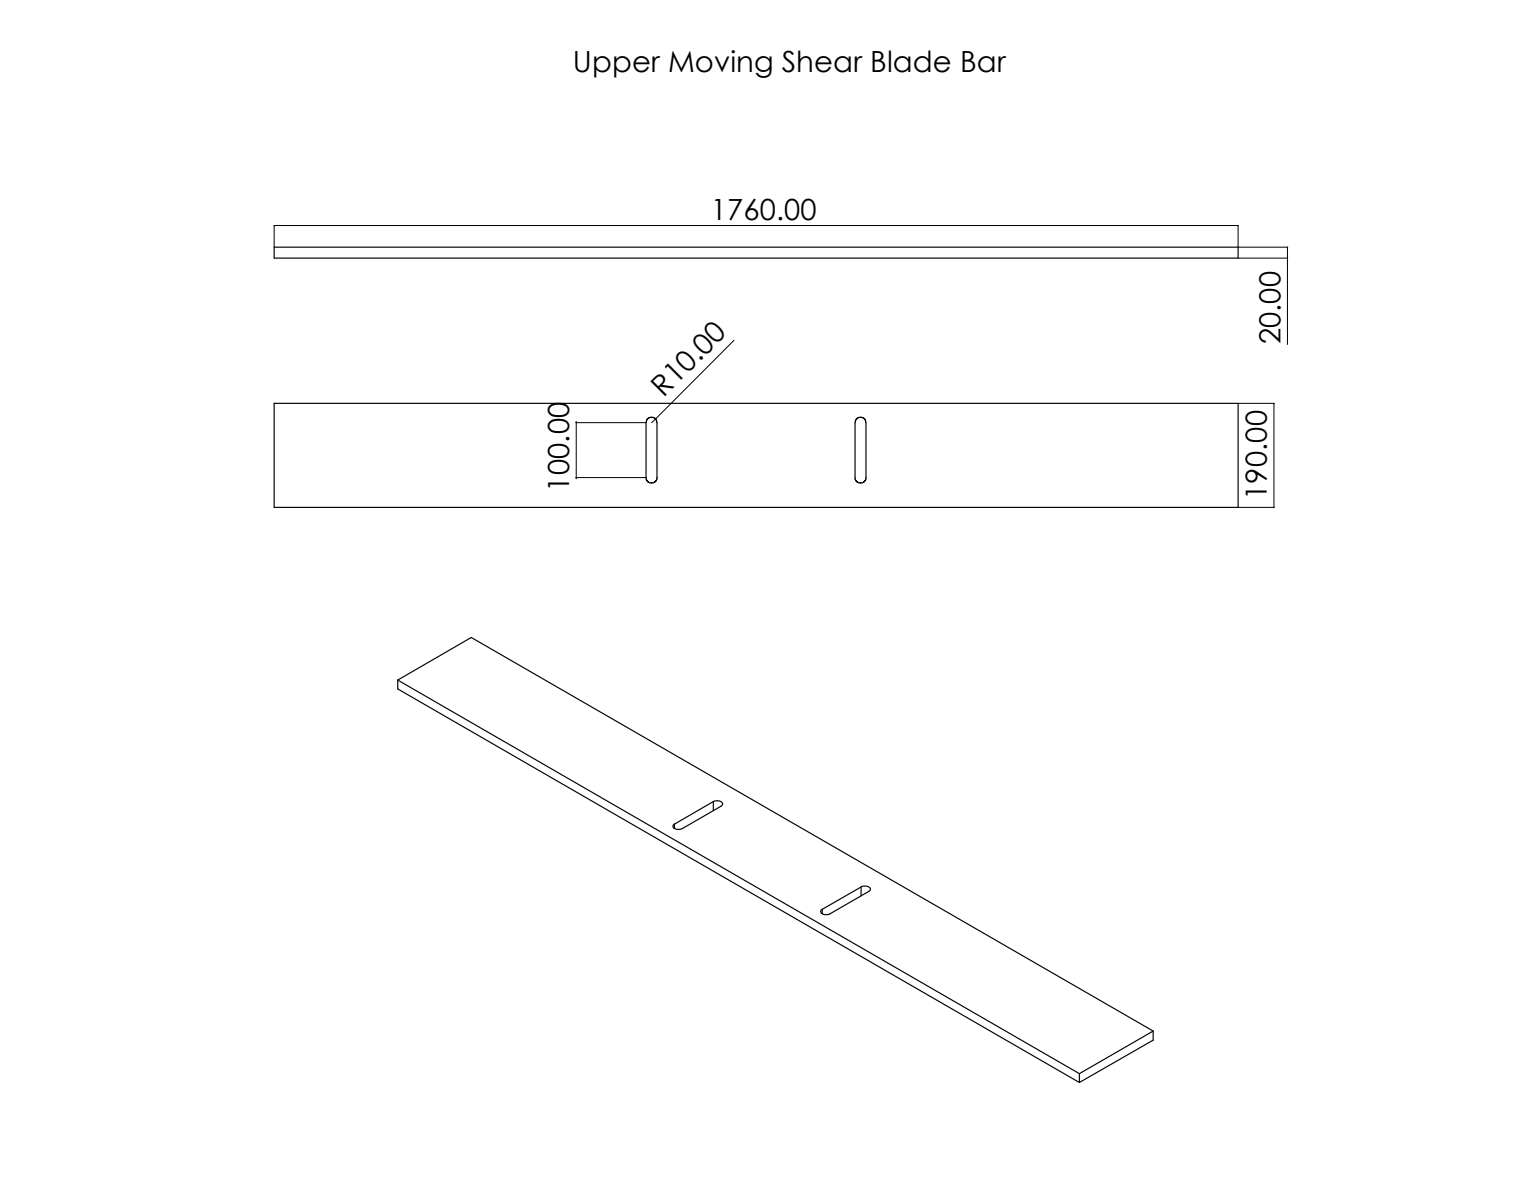
ISO-10303-21;
HEADER;
FILE_DESCRIPTION (('STEP AP214'),
    '1' );
FILE_NAME ('Upper Moving Shear Blade Bar.step',
    '2026-10-21T17:07:05',
    ( '' ),
    ( '' ),
    'SwSTEP 2.0',
    'SolidWorks 2025',
    '' );
FILE_SCHEMA (( 'AUTOMOTIVE_DESIGN' ));
ENDSEC;

DATA;
#27=ORIENTED_EDGE ( 'NONE', *, *, #22756, .F. ) ;
#29=LINE ( 'NONE', #5647, #43867 ) ;
#130=ORIENTED_EDGE ( 'NONE', *, *, #13131, .F. ) ;
#266=CARTESIAN_POINT ( 'NONE',  ( -180.7583438952258348, 394.6698570112193920, -224.9999999999999716 ) ) ;
#581=DIRECTION ( 'NONE',  ( 1.000000000000000000, -0.000000000000000000, 0.000000000000000000 ) ) ;
#901=DIRECTION ( 'NONE',  ( -1.000000000000000000, 1.892425610156518354E-16, 0.000000000000000000 ) ) ;
#935=DIRECTION ( 'NONE',  ( 1.000000000000000000, -8.326672684688676025E-16, 0.000000000000000000 ) ) ;
#1041=DIRECTION ( 'NONE',  ( -1.000000000000000000, 0.000000000000000000, 0.000000000000000000 ) ) ;
#1504=DIRECTION ( 'NONE',  ( 0.000000000000000000, 1.000000000000000000, 0.000000000000000000 ) ) ;
#1512=DIRECTION ( 'NONE',  ( 1.000000000000000000, 0.000000000000000000, -0.000000000000000000 ) ) ;
#1820=LINE ( 'NONE', #42339, #29283 ) ;
#1948=CARTESIAN_POINT ( 'NONE',  ( -190.7583438952259485, 394.6698570112193920, -274.9999999999999432 ) ) ;
#2119=LINE ( 'NONE', #11845, #11580 ) ;
#2127=FACE_OUTER_BOUND ( 'NONE', #44437, .T. ) ;
#2181=DIRECTION ( 'NONE',  ( 5.551115123125783688E-16, -1.000000000000000000, 0.000000000000000000 ) ) ;
#2576=EDGE_CURVE ( 'NONE', #42212, #45366, #43443, .T. ) ;
#2588=VECTOR ( 'NONE', #8913, 1000.000000000000000 ) ;
#2705=CARTESIAN_POINT ( 'NONE',  ( -180.7583438952258916, 294.6698570112193920, -224.9999999999999716 ) ) ;
#2814=ORIENTED_EDGE ( 'NONE', *, *, #20986, .T. ) ;
#2893=PLANE ( 'NONE',  #43166 ) ;
#2997=DIRECTION ( 'NONE',  ( 1.000000000000000000, 0.000000000000000000, 0.000000000000000000 ) ) ;
#3017=EDGE_CURVE ( 'NONE', #34587, #4508, #10696, .T. ) ;
#3213=ADVANCED_FACE ( 'NONE', ( #13857 ), #44817, .F. ) ;
#3240=VECTOR ( 'NONE', #38051, 1000.000000000000000 ) ;
#3278=DIRECTION ( 'NONE',  ( 8.326672684688676025E-16, -1.000000000000000000, 0.000000000000000000 ) ) ;
#3873=ORIENTED_EDGE ( 'NONE', *, *, #45007, .F. ) ;
#3881=PRODUCT_CONTEXT ( 'NONE', #32571, 'mechanical' ) ;
#3952=ADVANCED_BREP_SHAPE_REPRESENTATION ( '', ( #31868, #26858 ), #29006 ) ;
#4025=DIRECTION ( 'NONE',  ( -0.000000000000000000, -1.000000000000000000, -0.000000000000000000 ) ) ;
#4089=ADVANCED_FACE ( 'NONE', ( #39013 ), #14531, .F. ) ;
#4138=DIRECTION ( 'NONE',  ( -0.000000000000000000, -0.000000000000000000, 1.000000000000000000 ) ) ;
#4341=VERTEX_POINT ( 'NONE', #41669 ) ;
#4508=VERTEX_POINT ( 'NONE', #15438 ) ;
#4526=CARTESIAN_POINT ( 'NONE',  ( 200.7583438952258916, 294.6698570112193920, -274.9999999999999432 ) ) ;
#4681=DIRECTION ( 'NONE',  ( 1.000000000000000000, 0.000000000000000000, 0.000000000000000000 ) ) ;
#4964=EDGE_CURVE ( 'NONE', #45518, #8411, #15757, .T. ) ;
#5036=FACE_OUTER_BOUND ( 'NONE', #40726, .T. ) ;
#5163=ORIENTED_EDGE ( 'NONE', *, *, #18237, .F. ) ;
#5231=EDGE_LOOP ( 'NONE', ( #30202, #34802, #39527, #43738 ) ) ;
#5481=CIRCLE ( 'NONE', #32035, 10.00000000000006395 ) ;
#5489=VECTOR ( 'NONE', #4025, 1000.000000000000000 ) ;
#5504=EDGE_LOOP ( 'NONE', ( #24647, #14112, #14964, #44075 ) ) ;
#5520=DIRECTION ( 'NONE',  ( 1.000000000000000000, 0.000000000000000000, 0.000000000000000000 ) ) ;
#5588=STYLED_ITEM('',(#45779),#31868);
#5647=CARTESIAN_POINT ( 'NONE',  ( -200.7583438952257211, -1.114432678890474281E-13, -244.9999999999999716 ) ) ;
#5741=DIRECTION ( 'NONE',  ( 0.000000000000000000, -0.000000000000000000, 1.000000000000000000 ) ) ;
#5742=ORIENTED_EDGE ( 'NONE', *, *, #13885, .F. ) ;
#5789=EDGE_CURVE ( 'NONE', #17118, #17174, #27051, .T. ) ;
#5889=CARTESIAN_POINT ( 'NONE',  ( 200.7583438952259485, 394.6698570112193920, -274.9999999999999432 ) ) ;
#6035=ORIENTED_EDGE ( 'NONE', *, *, #39430, .F. ) ;
#6063=ORIENTED_EDGE ( 'NONE', *, *, #44462, .F. ) ;
#6075=DIRECTION ( 'NONE',  ( 1.000000000000000000, 0.000000000000000000, 0.000000000000000000 ) ) ;
#6252=AXIS2_PLACEMENT_3D ( 'NONE', #39369, #28745, #7499 ) ;
#6592=ORIENTED_EDGE ( 'NONE', *, *, #10942, .F. ) ;
#6658=EDGE_CURVE ( 'NONE', #34587, #37957, #36334, .T. ) ;
#6685=DIRECTION ( 'NONE',  ( 0.000000000000000000, -0.000000000000000000, 1.000000000000000000 ) ) ;
#6725=DIRECTION ( 'NONE',  ( -0.000000000000000000, -0.000000000000000000, 1.000000000000000000 ) ) ;
#6869=EDGE_LOOP ( 'NONE', ( #38404, #20507, #32932, #20169 ) ) ;
#6900=AXIS2_PLACEMENT_3D ( 'NONE', #21973, #935, #38668 ) ;
#7105=EDGE_LOOP ( 'NONE', ( #40674, #23927, #10024, #9838 ) ) ;
#7211=LINE ( 'NONE', #21284, #10700 ) ;
#7499=DIRECTION ( 'NONE',  ( 1.000000000000000000, 0.000000000000000000, 0.000000000000000000 ) ) ;
#7822=EDGE_CURVE ( 'NONE', #36156, #45518, #7211, .T. ) ;
#8396=CIRCLE ( 'NONE', #31234, 10.00000000000006395 ) ;
#8411=VERTEX_POINT ( 'NONE', #41123 ) ;
#8451=LINE ( 'NONE', #5889, #44550 ) ;
#8491=CARTESIAN_POINT ( 'NONE',  ( 200.7583438952259485, 394.6698570112193920, -244.9999999999999716 ) ) ;
#8510=CIRCLE ( 'NONE', #24705, 10.00000000000006395 ) ;
#8620=ORIENTED_EDGE ( 'NONE', *, *, #2576, .T. ) ;
#8685=CARTESIAN_POINT ( 'NONE',  ( 180.7583438952258348, 394.6698570112193920, -224.9999999999999716 ) ) ;
#8754=VERTEX_POINT ( 'NONE', #8491 ) ;
#8774=VERTEX_POINT ( 'NONE', #33871 ) ;
#8816=ORIENTED_EDGE ( 'NONE', *, *, #3017, .T. ) ;
#8860=ORIENTED_EDGE ( 'NONE', *, *, #2576, .F. ) ;
#8913=DIRECTION ( 'NONE',  ( 0.000000000000000000, 1.000000000000000000, 0.000000000000000000 ) ) ;
#9055=FACE_BOUND ( 'NONE', #27483, .T. ) ;
#9209=VERTEX_POINT ( 'NONE', #39869 ) ;
#9376=EDGE_CURVE ( 'NONE', #37957, #42212, #21806, .T. ) ;
#9394=AXIS2_PLACEMENT_3D ( 'NONE', #36836, #36620, #43534 ) ;
#9555=VERTEX_POINT ( 'NONE', #19060 ) ;
#9838=ORIENTED_EDGE ( 'NONE', *, *, #39646, .T. ) ;
#9993=( NAMED_UNIT ( * ) SI_UNIT ( $, .STERADIAN. ) SOLID_ANGLE_UNIT ( ) );
#10024=ORIENTED_EDGE ( 'NONE', *, *, #30379, .F. ) ;
#10532=CARTESIAN_POINT ( 'NONE',  ( -879.9999999999992042, 240.0000000000002274, -244.9999999999999716 ) ) ;
#10661=VECTOR ( 'NONE', #11122, 1000.000000000000000 ) ;
#10696=CIRCLE ( 'NONE', #18094, 10.00000000000000888 ) ;
#10700=VECTOR ( 'NONE', #35362, 1000.000000000000000 ) ;
#10730=FACE_OUTER_BOUND ( 'NONE', #45277, .T. ) ;
#10747=ORIENTED_EDGE ( 'NONE', *, *, #40559, .F. ) ;
#10942=EDGE_CURVE ( 'NONE', #32232, #4341, #17468, .T. ) ;
#11122=DIRECTION ( 'NONE',  ( 8.326672684688676025E-16, 1.000000000000000000, -0.000000000000000000 ) ) ;
#11149=( NAMED_UNIT ( * ) SI_UNIT ( $, .STERADIAN. ) SOLID_ANGLE_UNIT ( ) );
#11296=VECTOR ( 'NONE', #26217, 1000.000000000000000 ) ;
#11383=ORIENTED_EDGE ( 'NONE', *, *, #44462, .T. ) ;
#11412=DIRECTION ( 'NONE',  ( -0.000000000000000000, -0.000000000000000000, 1.000000000000000000 ) ) ;
#11440=ORIENTED_EDGE ( 'NONE', *, *, #38278, .F. ) ;
#11516=MECHANICAL_DESIGN_GEOMETRIC_PRESENTATION_REPRESENTATION('',(#5588),#17411);
#11580=VECTOR ( 'NONE', #16207, 1000.000000000000000 ) ;
#11627=DIRECTION ( 'NONE',  ( 1.000000000000000000, -5.551115123125783688E-16, 0.000000000000000000 ) ) ;
#11670=ADVANCED_FACE ( 'NONE', ( #19125 ), #33213, .F. ) ;
#11782=EDGE_LOOP ( 'NONE', ( #12503, #43387, #23339, #34195 ) ) ;
#11832=( LENGTH_UNIT ( ) NAMED_UNIT ( * ) SI_UNIT ( .MILLI., .METRE. ) );
#11845=CARTESIAN_POINT ( 'NONE',  ( -879.9999999999992042, 240.0000000000002274, -244.9999999999999716 ) ) ;
#11923=LINE ( 'NONE', #15614, #2588 ) ;
#12056=PRODUCT_DEFINITION_FORMATION_WITH_SPECIFIED_SOURCE ( 'ANY', '', #21473, .NOT_KNOWN. ) ;
#12153=VECTOR ( 'NONE', #14882, 1000.000000000000000 ) ;
#12380=FACE_BOUND ( 'NONE', #27839, .T. ) ;
#12503=ORIENTED_EDGE ( 'NONE', *, *, #17293, .T. ) ;
#12538=EDGE_CURVE ( 'NONE', #9209, #9555, #40081, .T. ) ;
#13131=EDGE_CURVE ( 'NONE', #4341, #27855, #26873, .T. ) ;
#13339=EDGE_CURVE ( 'NONE', #35556, #37602, #32944, .T. ) ;
#13644=ORIENTED_EDGE ( 'NONE', *, *, #39646, .F. ) ;
#13656=ORIENTED_EDGE ( 'NONE', *, *, #18237, .T. ) ;
#13662=ORIENTED_EDGE ( 'NONE', *, *, #19046, .T. ) ;
#13762=VECTOR ( 'NONE', #19614, 1000.000000000000000 ) ;
#13821=EDGE_LOOP ( 'NONE', ( #11383, #13644, #6035, #34359 ) ) ;
#13822=VECTOR ( 'NONE', #17631, 1000.000000000000000 ) ;
#13857=FACE_OUTER_BOUND ( 'NONE', #5231, .T. ) ;
#13885=EDGE_CURVE ( 'NONE', #4508, #35556, #1820, .T. ) ;
#13911=LINE ( 'NONE', #35366, #39751 ) ;
#14064=ORIENTED_EDGE ( 'NONE', *, *, #21274, .F. ) ;
#14112=ORIENTED_EDGE ( 'NONE', *, *, #42969, .T. ) ;
#14140=VECTOR ( 'NONE', #34457, 1000.000000000000000 ) ;
#14164=VERTEX_POINT ( 'NONE', #40195 ) ;
#14466=DIRECTION ( 'NONE',  ( 0.000000000000000000, 0.000000000000000000, 1.000000000000000000 ) ) ;
#14475=CARTESIAN_POINT ( 'NONE',  ( 879.9999999999992042, 239.9999999999998863, -244.9999999999999716 ) ) ;
#14531=PLANE ( 'NONE',  #44652 ) ;
#14871=ADVANCED_FACE ( 'NONE', ( #5036 ), #33215, .T. ) ;
#14877=LINE ( 'NONE', #25712, #23876 ) ;
#14882=DIRECTION ( 'NONE',  ( -0.000000000000000000, -0.000000000000000000, 1.000000000000000000 ) ) ;
#14964=ORIENTED_EDGE ( 'NONE', *, *, #24944, .F. ) ;
#15080=ORIENTED_EDGE ( 'NONE', *, *, #13885, .T. ) ;
#15325=CARTESIAN_POINT ( 'NONE',  ( 879.9999999999992042, 429.9999999999999432, -224.9999999999999716 ) ) ;
#15377=ORIENTED_EDGE ( 'NONE', *, *, #38278, .T. ) ;
#15398=FACE_BOUND ( 'NONE', #24156, .T. ) ;
#15438=CARTESIAN_POINT ( 'NONE',  ( -180.7583438952258916, 294.6698570112193920, -244.9999999999999716 ) ) ;
#15562=CARTESIAN_POINT ( 'NONE',  ( 180.7583438952258348, 394.6698570112193920, -274.9999999999999432 ) ) ;
#15614=CARTESIAN_POINT ( 'NONE',  ( -879.9999999999992042, 240.0000000000002274, -244.9999999999999716 ) ) ;
#15757=LINE ( 'NONE', #15325, #30675 ) ;
#15973=AXIS2_PLACEMENT_3D ( 'NONE', #26377, #16206, #4681 ) ;
#16073=EDGE_LOOP ( 'NONE', ( #44536, #19765, #44906, #31596 ) ) ;
#16206=DIRECTION ( 'NONE',  ( 0.000000000000000000, 0.000000000000000000, 1.000000000000000000 ) ) ;
#16207=DIRECTION ( 'NONE',  ( -0.000000000000000000, -0.000000000000000000, 1.000000000000000000 ) ) ;
#16215=CARTESIAN_POINT ( 'NONE',  ( 0.000000000000000000, 0.000000000000000000, -224.9999999999999716 ) ) ;
#16361=ORIENTED_EDGE ( 'NONE', *, *, #9376, .F. ) ;
#16538=ORIENTED_EDGE ( 'NONE', *, *, #17293, .F. ) ;
#16714=ORIENTED_EDGE ( 'NONE', *, *, #45007, .T. ) ;
#16743=AXIS2_PLACEMENT_3D ( 'NONE', #29730, #43808, #40385 ) ;
#16824=ORIENTED_EDGE ( 'NONE', *, *, #13339, .F. ) ;
#17054=ADVANCED_FACE ( 'NONE', ( #43935, #9055, #2127 ), #23121, .T. ) ;
#17118=VERTEX_POINT ( 'NONE', #43706 ) ;
#17125=FACE_OUTER_BOUND ( 'NONE', #41293, .T. ) ;
#17174=VERTEX_POINT ( 'NONE', #19016 ) ;
#17293=EDGE_CURVE ( 'NONE', #45518, #9555, #20361, .T. ) ;
#17411=( GEOMETRIC_REPRESENTATION_CONTEXT ( 3 ) GLOBAL_UNCERTAINTY_ASSIGNED_CONTEXT ( ( #32911 ) ) GLOBAL_UNIT_ASSIGNED_CONTEXT ( ( #37939, #45108, #9993 ) ) REPRESENTATION_CONTEXT ( 'NONE', 'WORKASPACE' ) );
#17417=PRODUCT_DEFINITION_SHAPE ( 'NONE', 'NONE',  #44518 ) ;
#17429=PLANE ( 'NONE',  #6900 ) ;
#17468=CIRCLE ( 'NONE', #15973, 10.00000000000000888 ) ;
#17487=LINE ( 'NONE', #28557, #45401 ) ;
#17631=DIRECTION ( 'NONE',  ( -0.000000000000000000, -0.000000000000000000, 1.000000000000000000 ) ) ;
#17673=CARTESIAN_POINT ( 'NONE',  ( 879.9999999999992042, 239.9999999999998863, -244.9999999999999716 ) ) ;
#17721=LINE ( 'NONE', #34343, #33434 ) ;
#17749=ORIENTED_EDGE ( 'NONE', *, *, #7822, .T. ) ;
#18085=( NAMED_UNIT ( * ) PLANE_ANGLE_UNIT ( ) SI_UNIT ( $, .RADIAN. ) );
#18094=AXIS2_PLACEMENT_3D ( 'NONE', #27933, #6685, #30948 ) ;
#18237=EDGE_CURVE ( 'NONE', #45366, #8774, #8510, .T. ) ;
#18305=CARTESIAN_POINT ( 'NONE',  ( -200.7583438952259485, 394.6698570112193920, -244.9999999999999716 ) ) ;
#18374=FACE_OUTER_BOUND ( 'NONE', #7105, .T. ) ;
#18435=VERTEX_POINT ( 'NONE', #10532 ) ;
#18482=EDGE_CURVE ( 'NONE', #8774, #37957, #17487, .T. ) ;
#18558=DIRECTION ( 'NONE',  ( -1.000000000000000000, 1.892425610156518354E-16, 0.000000000000000000 ) ) ;
#18766=EDGE_CURVE ( 'NONE', #17174, #4341, #29464, .T. ) ;
#18950=AXIS2_PLACEMENT_3D ( 'NONE', #20983, #35079, #43391 ) ;
#19016=CARTESIAN_POINT ( 'NONE',  ( 200.7583438952258916, 294.6698570112193920, -244.9999999999999716 ) ) ;
#19046=EDGE_CURVE ( 'NONE', #37602, #34587, #29, .T. ) ;
#19060=CARTESIAN_POINT ( 'NONE',  ( 879.9999999999992042, 239.9999999999998863, -224.9999999999999716 ) ) ;
#19064=CARTESIAN_POINT ( 'NONE',  ( -190.7583438952259485, 394.6698570112193920, -244.9999999999999716 ) ) ;
#19086=ADVANCED_FACE ( 'NONE', ( #17125 ), #27747, .F. ) ;
#19125=FACE_OUTER_BOUND ( 'NONE', #6869, .T. ) ;
#19223=DIRECTION ( 'NONE',  ( 0.000000000000000000, 0.000000000000000000, -1.000000000000000000 ) ) ;
#19374=ORIENTED_EDGE ( 'NONE', *, *, #18482, .F. ) ;
#19492=DIRECTION ( 'NONE',  ( 0.000000000000000000, -0.000000000000000000, 1.000000000000000000 ) ) ;
#19500=DIRECTION ( 'NONE',  ( 1.000000000000000000, 0.000000000000000000, 0.000000000000000000 ) ) ;
#19614=DIRECTION ( 'NONE',  ( -0.000000000000000000, -0.000000000000000000, 1.000000000000000000 ) ) ;
#19738=PLANE ( 'NONE',  #9394 ) ;
#19765=ORIENTED_EDGE ( 'NONE', *, *, #18482, .T. ) ;
#20169=ORIENTED_EDGE ( 'NONE', *, *, #3017, .F. ) ;
#20361=LINE ( 'NONE', #34683, #14140 ) ;
#20444=CARTESIAN_POINT ( 'NONE',  ( 879.9999999999992042, 239.9999999999998863, -244.9999999999999716 ) ) ;
#20507=ORIENTED_EDGE ( 'NONE', *, *, #9376, .T. ) ;
#20518=ADVANCED_FACE ( 'NONE', ( #15398, #12380, #43551 ), #26457, .F. ) ;
#20563=PRODUCT_DEFINITION_CONTEXT ( 'detailed design', #38789, 'design' ) ;
#20649=CARTESIAN_POINT ( 'NONE',  ( 879.9999999999992042, 429.9999999999999432, -224.9999999999999716 ) ) ;
#20659=DIRECTION ( 'NONE',  ( -1.000000000000000000, 1.892425610156518601E-16, 0.000000000000000000 ) ) ;
#20706=CARTESIAN_POINT ( 'NONE',  ( -879.9999999999992042, 430.0000000000002842, -224.9999999999999716 ) ) ;
#20878=CARTESIAN_POINT ( 'NONE',  ( 879.9999999999992042, 239.9999999999998863, -244.9999999999999716 ) ) ;
#20983=CARTESIAN_POINT ( 'NONE',  ( 190.7583438952258916, 294.6698570112193920, -244.9999999999999716 ) ) ;
#20986=EDGE_CURVE ( 'NONE', #8411, #9209, #45626, .T. ) ;
#21034=ADVANCED_FACE ( 'NONE', ( #32442 ), #25258, .F. ) ;
#21192=ORIENTED_EDGE ( 'NONE', *, *, #28021, .T. ) ;
#21250=ADVANCED_FACE ( 'NONE', ( #10730 ), #38930, .F. ) ;
#21274=EDGE_CURVE ( 'NONE', #37602, #8774, #31958, .T. ) ;
#21284=CARTESIAN_POINT ( 'NONE',  ( -879.9999999999992042, 430.0000000000002842, -224.9999999999999716 ) ) ;
#21301=LINE ( 'NONE', #29092, #35871 ) ;
#21331=DIRECTION ( 'NONE',  ( 8.326672684688676025E-16, 1.000000000000000000, 0.000000000000000000 ) ) ;
#21386=CARTESIAN_POINT ( 'NONE',  ( 180.7583438952258348, 394.6698570112193920, -244.9999999999999716 ) ) ;
#21396=DIRECTION ( 'NONE',  ( 5.551115123125783688E-16, -1.000000000000000000, 0.000000000000000000 ) ) ;
#21473=PRODUCT ( 'Upper Moving Shear Blade Bar', 'Upper Moving Shear Blade Bar', '', ( #3881 ) ) ;
#21555=DIRECTION ( 'NONE',  ( 0.000000000000000000, 0.000000000000000000, 1.000000000000000000 ) ) ;
#21806=CIRCLE ( 'NONE', #27706, 10.00000000000000888 ) ;
#21973=CARTESIAN_POINT ( 'NONE',  ( -180.7583438952258348, 394.6698570112193920, -274.9999999999999432 ) ) ;
#22096=ADVANCED_FACE ( 'NONE', ( #28051 ), #2893, .F. ) ;
#22217=EDGE_LOOP ( 'NONE', ( #43972, #8620, #28755, #5742 ) ) ;
#22261=PLANE ( 'NONE',  #32282 ) ;
#22756=EDGE_CURVE ( 'NONE', #23583, #14164, #37016, .T. ) ;
#23121=PLANE ( 'NONE',  #25898 ) ;
#23153=CARTESIAN_POINT ( 'NONE',  ( 0.000000000000000000, 0.000000000000000000, 0.000000000000000000 ) ) ;
#23221=AXIS2_PLACEMENT_3D ( 'NONE', #1948, #6725, #19500 ) ;
#23299=LINE ( 'NONE', #37620, #13762 ) ;
#23339=ORIENTED_EDGE ( 'NONE', *, *, #20986, .F. ) ;
#23583=VERTEX_POINT ( 'NONE', #21386 ) ;
#23876=VECTOR ( 'NONE', #21555, 1000.000000000000000 ) ;
#23927=ORIENTED_EDGE ( 'NONE', *, *, #28021, .F. ) ;
#23931=CARTESIAN_POINT ( 'NONE',  ( 879.9999999999992042, 239.9999999999998863, -224.9999999999999716 ) ) ;
#23948=VECTOR ( 'NONE', #11412, 1000.000000000000000 ) ;
#24137=ORIENTED_EDGE ( 'NONE', *, *, #39430, .T. ) ;
#24156=EDGE_LOOP ( 'NONE', ( #15377, #34878, #36680, #27894 ) ) ;
#24529=EDGE_LOOP ( 'NONE', ( #10747, #130, #6592, #27288 ) ) ;
#24566=DIRECTION ( 'NONE',  ( -1.000000000000000000, 0.000000000000000000, 0.000000000000000000 ) ) ;
#24647=ORIENTED_EDGE ( 'NONE', *, *, #22756, .T. ) ;
#24705=AXIS2_PLACEMENT_3D ( 'NONE', #30943, #28096, #35257 ) ;
#24785=PLANE ( 'NONE',  #27257 ) ;
#24834=ORIENTED_EDGE ( 'NONE', *, *, #13339, .T. ) ;
#24944=EDGE_CURVE ( 'NONE', #17118, #32232, #23299, .T. ) ;
#25258=PLANE ( 'NONE',  #35040 ) ;
#25472=CARTESIAN_POINT ( 'NONE',  ( 200.7583438952259485, 394.6698570112193920, -274.9999999999999432 ) ) ;
#25712=CARTESIAN_POINT ( 'NONE',  ( -879.9999999999992042, 430.0000000000002842, -244.9999999999999716 ) ) ;
#25898=AXIS2_PLACEMENT_3D ( 'NONE', #16215, #37226, #26600 ) ;
#25942=DIRECTION ( 'NONE',  ( -0.000000000000000000, -0.000000000000000000, 1.000000000000000000 ) ) ;
#26205=VECTOR ( 'NONE', #25942, 1000.000000000000000 ) ;
#26217=DIRECTION ( 'NONE',  ( 8.326672684688676025E-16, -1.000000000000000000, 0.000000000000000000 ) ) ;
#26377=CARTESIAN_POINT ( 'NONE',  ( 190.7583438952258916, 294.6698570112193920, -224.9999999999999716 ) ) ;
#26457=PLANE ( 'NONE',  #34231 ) ;
#26600=DIRECTION ( 'NONE',  ( 1.000000000000000000, 0.000000000000000000, -0.000000000000000000 ) ) ;
#26858=AXIS2_PLACEMENT_3D ( 'NONE', #23153, #34241, #6075 ) ;
#26873=LINE ( 'NONE', #33359, #27021 ) ;
#26975=ADVANCED_FACE ( 'NONE', ( #34042 ), #19738, .F. ) ;
#27021=VECTOR ( 'NONE', #33590, 1000.000000000000000 ) ;
#27051=CIRCLE ( 'NONE', #18950, 10.00000000000000888 ) ;
#27257=AXIS2_PLACEMENT_3D ( 'NONE', #25472, #11627, #35874 ) ;
#27288=ORIENTED_EDGE ( 'NONE', *, *, #42969, .F. ) ;
#27327=CARTESIAN_POINT ( 'NONE',  ( -200.7583438952258916, 294.6698570112193920, -244.9999999999999716 ) ) ;
#27474=LINE ( 'NONE', #34858, #36099 ) ;
#27483=EDGE_LOOP ( 'NONE', ( #5163, #8860, #16361, #19374 ) ) ;
#27706=AXIS2_PLACEMENT_3D ( 'NONE', #32694, #14466, #1041 ) ;
#27747=CYLINDRICAL_SURFACE ( 'NONE', #23221, 10.00000000000006395 ) ;
#27839=EDGE_LOOP ( 'NONE', ( #15080, #24834, #13662, #8816 ) ) ;
#27855=VERTEX_POINT ( 'NONE', #36329 ) ;
#27894=ORIENTED_EDGE ( 'NONE', *, *, #5789, .T. ) ;
#27933=CARTESIAN_POINT ( 'NONE',  ( -190.7583438952258916, 294.6698570112193920, -244.9999999999999716 ) ) ;
#28021=EDGE_CURVE ( 'NONE', #39568, #36156, #14877, .T. ) ;
#28051=FACE_OUTER_BOUND ( 'NONE', #13821, .T. ) ;
#28096=DIRECTION ( 'NONE',  ( 0.000000000000000000, 0.000000000000000000, 1.000000000000000000 ) ) ;
#28157=DIRECTION ( 'NONE',  ( -0.000000000000000000, -0.000000000000000000, 1.000000000000000000 ) ) ;
#28527=DIRECTION ( 'NONE',  ( 0.000000000000000000, 0.000000000000000000, -1.000000000000000000 ) ) ;
#28557=CARTESIAN_POINT ( 'NONE',  ( -200.7583438952259485, 394.6698570112193920, -224.9999999999999716 ) ) ;
#28677=EDGE_CURVE ( 'NONE', #8754, #23583, #5481, .T. ) ;
#28724=LINE ( 'NONE', #32421, #39617 ) ;
#28745=DIRECTION ( 'NONE',  ( -0.000000000000000000, -0.000000000000000000, 1.000000000000000000 ) ) ;
#28755=ORIENTED_EDGE ( 'NONE', *, *, #34585, .F. ) ;
#29006=( GEOMETRIC_REPRESENTATION_CONTEXT ( 3 ) GLOBAL_UNCERTAINTY_ASSIGNED_CONTEXT ( ( #34873 ) ) GLOBAL_UNIT_ASSIGNED_CONTEXT ( ( #11832, #18085, #11149 ) ) REPRESENTATION_CONTEXT ( 'NONE', 'WORKASPACE' ) );
#29092=CARTESIAN_POINT ( 'NONE',  ( 879.9999999999992042, 429.9999999999999432, -244.9999999999999716 ) ) ;
#29128=CLOSED_SHELL ( 'NONE', ( #21034, #22096, #33971, #20518, #17054, #14871, #19086, #43542, #11670, #4089, #21250, #39277, #3213, #26975 ) ) ;
#29272=ORIENTED_EDGE ( 'NONE', *, *, #13131, .T. ) ;
#29283=VECTOR ( 'NONE', #21331, 1000.000000000000000 ) ;
#29285=AXIS2_PLACEMENT_3D ( 'NONE', #35759, #4138, #32306 ) ;
#29464=LINE ( 'NONE', #4526, #33555 ) ;
#29691=CARTESIAN_POINT ( 'NONE',  ( 0.000000000000000000, 0.000000000000000000, -244.9999999999999716 ) ) ;
#29730=CARTESIAN_POINT ( 'NONE',  ( 8.137430123673030402E-14, 430.0000000000000568, 0.000000000000000000 ) ) ;
#29994=DIRECTION ( 'NONE',  ( 1.000000000000000000, 0.000000000000000000, 0.000000000000000000 ) ) ;
#30035=CARTESIAN_POINT ( 'NONE',  ( -200.7583438952258916, 294.6698570112193920, -224.9999999999999716 ) ) ;
#30202=ORIENTED_EDGE ( 'NONE', *, *, #24944, .T. ) ;
#30379=EDGE_CURVE ( 'NONE', #18435, #39568, #11923, .T. ) ;
#30675=VECTOR ( 'NONE', #19223, 1000.000000000000000 ) ;
#30718=AXIS2_PLACEMENT_3D ( 'NONE', #19064, #19492, #43982 ) ;
#30943=CARTESIAN_POINT ( 'NONE',  ( -190.7583438952259485, 394.6698570112193920, -224.9999999999999716 ) ) ;
#30948=DIRECTION ( 'NONE',  ( 1.000000000000000000, 0.000000000000000000, 0.000000000000000000 ) ) ;
#30969=CARTESIAN_POINT ( 'NONE',  ( -180.7583438952258348, 394.6698570112193920, -244.9999999999999716 ) ) ;
#31234=AXIS2_PLACEMENT_3D ( 'NONE', #35568, #32359, #5520 ) ;
#31596=ORIENTED_EDGE ( 'NONE', *, *, #19046, .F. ) ;
#31735=DIRECTION ( 'NONE',  ( 0.000000000000000000, 0.000000000000000000, 1.000000000000000000 ) ) ;
#31868=MANIFOLD_SOLID_BREP ( 'Cut-Extrude5[2]', #29128 ) ;
#31958=LINE ( 'NONE', #43050, #23948 ) ;
#32035=AXIS2_PLACEMENT_3D ( 'NONE', #33456, #5741, #29994 ) ;
#32167=SHAPE_REPRESENTATION_RELATIONSHIP ( 'NONE' , 'NONE' ,  #36841, #3952 ) ;
#32168=VECTOR ( 'NONE', #35697, 1000.000000000000000 ) ;
#32221=CARTESIAN_POINT ( 'NONE',  ( -879.9999999999992042, 240.0000000000002274, -244.9999999999999716 ) ) ;
#32232=VERTEX_POINT ( 'NONE', #43622 ) ;
#32282=AXIS2_PLACEMENT_3D ( 'NONE', #32221, #581, #28527 ) ;
#32302=DIRECTION ( 'NONE',  ( 5.551115123125783688E-16, -1.000000000000000000, 0.000000000000000000 ) ) ;
#32306=DIRECTION ( 'NONE',  ( 1.000000000000000000, 0.000000000000000000, 0.000000000000000000 ) ) ;
#32345=EDGE_CURVE ( 'NONE', #8411, #39568, #21301, .T. ) ;
#32359=DIRECTION ( 'NONE',  ( 0.000000000000000000, 0.000000000000000000, 1.000000000000000000 ) ) ;
#32421=CARTESIAN_POINT ( 'NONE',  ( 879.9999999999992042, 239.9999999999998863, -244.9999999999999716 ) ) ;
#32433=CARTESIAN_POINT ( 'NONE',  ( -200.7583438952258916, 294.6698570112193920, -274.9999999999999432 ) ) ;
#32442=FACE_OUTER_BOUND ( 'NONE', #11782, .T. ) ;
#32571=APPLICATION_CONTEXT ( 'automotive_design' ) ;
#32694=CARTESIAN_POINT ( 'NONE',  ( -190.7583438952258916, 294.6698570112193920, -224.9999999999999716 ) ) ;
#32911=UNCERTAINTY_MEASURE_WITH_UNIT (LENGTH_MEASURE( 1.000000000000000082E-05 ), #37939, 'distance_accuracy_value', 'NONE');
#32932=ORIENTED_EDGE ( 'NONE', *, *, #44199, .F. ) ;
#32944=CIRCLE ( 'NONE', #30718, 10.00000000000006395 ) ;
#33168=CARTESIAN_POINT ( 'NONE',  ( -879.9999999999992042, 240.0000000000002274, -224.9999999999999716 ) ) ;
#33213=CYLINDRICAL_SURFACE ( 'NONE', #29285, 10.00000000000000888 ) ;
#33215=PLANE ( 'NONE',  #16743 ) ;
#33359=CARTESIAN_POINT ( 'NONE',  ( 200.7583438952259485, 394.6698570112193920, -224.9999999999999716 ) ) ;
#33365=DIRECTION ( 'NONE',  ( -0.000000000000000000, -0.000000000000000000, 1.000000000000000000 ) ) ;
#33434=VECTOR ( 'NONE', #37814, 1000.000000000000000 ) ;
#33456=CARTESIAN_POINT ( 'NONE',  ( 190.7583438952259485, 394.6698570112193920, -244.9999999999999716 ) ) ;
#33555=VECTOR ( 'NONE', #33365, 1000.000000000000000 ) ;
#33590=DIRECTION ( 'NONE',  ( 5.551115123125783688E-16, 1.000000000000000000, -0.000000000000000000 ) ) ;
#33871=CARTESIAN_POINT ( 'NONE',  ( -200.7583438952259485, 394.6698570112193920, -224.9999999999999716 ) ) ;
#33912=ORIENTED_EDGE ( 'NONE', *, *, #32345, .T. ) ;
#33971=ADVANCED_FACE ( 'NONE', ( #18374 ), #22261, .F. ) ;
#34042=FACE_OUTER_BOUND ( 'NONE', #5504, .T. ) ;
#34195=ORIENTED_EDGE ( 'NONE', *, *, #4964, .F. ) ;
#34231=AXIS2_PLACEMENT_3D ( 'NONE', #29691, #40558, #1512 ) ;
#34241=DIRECTION ( 'NONE',  ( 0.000000000000000000, 0.000000000000000000, 1.000000000000000000 ) ) ;
#34343=CARTESIAN_POINT ( 'NONE',  ( -180.7583438952258916, 294.6698570112193920, -274.9999999999999432 ) ) ;
#34359=ORIENTED_EDGE ( 'NONE', *, *, #12538, .T. ) ;
#34457=DIRECTION ( 'NONE',  ( -0.000000000000000000, -1.000000000000000000, -0.000000000000000000 ) ) ;
#34487=LINE ( 'NONE', #38639, #13822 ) ;
#34585=EDGE_CURVE ( 'NONE', #35556, #45366, #34487, .T. ) ;
#34587=VERTEX_POINT ( 'NONE', #27327 ) ;
#34640=CARTESIAN_POINT ( 'NONE',  ( 190.7583438952258916, 294.6698570112193920, -274.9999999999999432 ) ) ;
#34683=CARTESIAN_POINT ( 'NONE',  ( 879.9999999999992042, 239.9999999999998863, -224.9999999999999716 ) ) ;
#34802=ORIENTED_EDGE ( 'NONE', *, *, #10942, .T. ) ;
#34858=CARTESIAN_POINT ( 'NONE',  ( 200.7583438952257211, -1.114432678890474281E-13, -244.9999999999999716 ) ) ;
#34873=UNCERTAINTY_MEASURE_WITH_UNIT (LENGTH_MEASURE( 1.000000000000000082E-05 ), #11832, 'distance_accuracy_value', 'NONE');
#34878=ORIENTED_EDGE ( 'NONE', *, *, #28677, .T. ) ;
#34954=VECTOR ( 'NONE', #1504, 1000.000000000000000 ) ;
#35040=AXIS2_PLACEMENT_3D ( 'NONE', #17673, #24566, #31735 ) ;
#35079=DIRECTION ( 'NONE',  ( 0.000000000000000000, -0.000000000000000000, 1.000000000000000000 ) ) ;
#35257=DIRECTION ( 'NONE',  ( -1.000000000000000000, 0.000000000000000000, 0.000000000000000000 ) ) ;
#35362=DIRECTION ( 'NONE',  ( 1.000000000000000000, -1.892425610156518354E-16, 0.000000000000000000 ) ) ;
#35366=CARTESIAN_POINT ( 'NONE',  ( 180.7583438952261474, 1.505115564641941601E-13, -244.9999999999999716 ) ) ;
#35556=VERTEX_POINT ( 'NONE', #30969 ) ;
#35568=CARTESIAN_POINT ( 'NONE',  ( 190.7583438952259485, 394.6698570112193920, -224.9999999999999716 ) ) ;
#35697=DIRECTION ( 'NONE',  ( -0.000000000000000000, -0.000000000000000000, 1.000000000000000000 ) ) ;
#35759=CARTESIAN_POINT ( 'NONE',  ( -190.7583438952258916, 294.6698570112193920, -274.9999999999999432 ) ) ;
#35871=VECTOR ( 'NONE', #901, 1000.000000000000000 ) ;
#35874=DIRECTION ( 'NONE',  ( 5.551115123125783688E-16, 1.000000000000000000, 0.000000000000000000 ) ) ;
#35992=DIRECTION ( 'NONE',  ( -1.000000000000000000, -5.551115123125783688E-16, 0.000000000000000000 ) ) ;
#36099=VECTOR ( 'NONE', #38119, 1000.000000000000000 ) ;
#36156=VERTEX_POINT ( 'NONE', #20706 ) ;
#36329=CARTESIAN_POINT ( 'NONE',  ( 200.7583438952259485, 394.6698570112193920, -224.9999999999999716 ) ) ;
#36334=LINE ( 'NONE', #32433, #12153 ) ;
#36620=DIRECTION ( 'NONE',  ( -1.000000000000000000, -8.326672684688676025E-16, 0.000000000000000000 ) ) ;
#36632=LINE ( 'NONE', #33168, #34954 ) ;
#36680=ORIENTED_EDGE ( 'NONE', *, *, #37114, .T. ) ;
#36836=CARTESIAN_POINT ( 'NONE',  ( 180.7583438952258348, 394.6698570112193920, -274.9999999999999432 ) ) ;
#36841=SHAPE_REPRESENTATION ( 'Upper Moving Shear Blade Bar', ( #26858 ), #29006 ) ;
#37016=LINE ( 'NONE', #15562, #26205 ) ;
#37114=EDGE_CURVE ( 'NONE', #23583, #17118, #13911, .T. ) ;
#37226=DIRECTION ( 'NONE',  ( 0.000000000000000000, -0.000000000000000000, 1.000000000000000000 ) ) ;
#37602=VERTEX_POINT ( 'NONE', #18305 ) ;
#37620=CARTESIAN_POINT ( 'NONE',  ( 180.7583438952258916, 294.6698570112193920, -274.9999999999999432 ) ) ;
#37814=DIRECTION ( 'NONE',  ( -0.000000000000000000, -0.000000000000000000, 1.000000000000000000 ) ) ;
#37939=( LENGTH_UNIT ( ) NAMED_UNIT ( * ) SI_UNIT ( .MILLI., .METRE. ) );
#37957=VERTEX_POINT ( 'NONE', #30035 ) ;
#38051=DIRECTION ( 'NONE',  ( -1.000000000000000000, 1.892425610156518354E-16, 0.000000000000000000 ) ) ;
#38119=DIRECTION ( 'NONE',  ( 5.551115123125783688E-16, 1.000000000000000000, 0.000000000000000000 ) ) ;
#38235=DIRECTION ( 'NONE',  ( 1.892425610156518601E-16, 1.000000000000000000, 0.000000000000000000 ) ) ;
#38278=EDGE_CURVE ( 'NONE', #17174, #8754, #27474, .T. ) ;
#38404=ORIENTED_EDGE ( 'NONE', *, *, #6658, .T. ) ;
#38443=CARTESIAN_POINT ( 'NONE',  ( -180.7583438952258348, 394.6698570112193920, -224.9999999999999716 ) ) ;
#38573=ORIENTED_EDGE ( 'NONE', *, *, #40559, .T. ) ;
#38639=CARTESIAN_POINT ( 'NONE',  ( -180.7583438952258348, 394.6698570112193920, -274.9999999999999432 ) ) ;
#38668=DIRECTION ( 'NONE',  ( 8.326672684688676025E-16, 1.000000000000000000, 0.000000000000000000 ) ) ;
#38789=APPLICATION_CONTEXT ( 'automotive_design' ) ;
#38930=CYLINDRICAL_SURFACE ( 'NONE', #6252, 10.00000000000006395 ) ;
#39013=FACE_OUTER_BOUND ( 'NONE', #16073, .T. ) ;
#39055=ORIENTED_EDGE ( 'NONE', *, *, #28677, .F. ) ;
#39225=SHAPE_DEFINITION_REPRESENTATION ( #17417, #36841 ) ;
#39277=ADVANCED_FACE ( 'NONE', ( #39817 ), #24785, .F. ) ;
#39369=CARTESIAN_POINT ( 'NONE',  ( 190.7583438952259485, 394.6698570112193920, -274.9999999999999432 ) ) ;
#39430=EDGE_CURVE ( 'NONE', #9209, #18435, #28724, .T. ) ;
#39527=ORIENTED_EDGE ( 'NONE', *, *, #18766, .F. ) ;
#39568=VERTEX_POINT ( 'NONE', #40026 ) ;
#39617=VECTOR ( 'NONE', #18558, 1000.000000000000000 ) ;
#39646=EDGE_CURVE ( 'NONE', #18435, #44320, #2119, .T. ) ;
#39695=ORIENTED_EDGE ( 'NONE', *, *, #18766, .T. ) ;
#39709=CARTESIAN_POINT ( 'NONE',  ( -200.7583438952259485, 394.6698570112193920, -274.9999999999999432 ) ) ;
#39751=VECTOR ( 'NONE', #3278, 1000.000000000000000 ) ;
#39817=FACE_OUTER_BOUND ( 'NONE', #44679, .T. ) ;
#39869=CARTESIAN_POINT ( 'NONE',  ( 879.9999999999992042, 239.9999999999998863, -244.9999999999999716 ) ) ;
#39970=EDGE_LOOP ( 'NONE', ( #2814, #24137, #43514, #40967 ) ) ;
#40026=CARTESIAN_POINT ( 'NONE',  ( -879.9999999999992042, 430.0000000000002842, -244.9999999999999716 ) ) ;
#40081=LINE ( 'NONE', #14475, #32168 ) ;
#40195=CARTESIAN_POINT ( 'NONE',  ( 180.7583438952258348, 394.6698570112193920, -224.9999999999999716 ) ) ;
#40385=DIRECTION ( 'NONE',  ( -1.000000000000000000, 1.892425610156518354E-16, 0.000000000000000000 ) ) ;
#40558=DIRECTION ( 'NONE',  ( 0.000000000000000000, -0.000000000000000000, 1.000000000000000000 ) ) ;
#40559=EDGE_CURVE ( 'NONE', #27855, #14164, #8396, .T. ) ;
#40674=ORIENTED_EDGE ( 'NONE', *, *, #45098, .T. ) ;
#40726=EDGE_LOOP ( 'NONE', ( #21192, #17749, #45008, #33912 ) ) ;
#40925=AXIS2_PLACEMENT_3D ( 'NONE', #34640, #28157, #2997 ) ;
#40967=ORIENTED_EDGE ( 'NONE', *, *, #32345, .F. ) ;
#41123=CARTESIAN_POINT ( 'NONE',  ( 879.9999999999992042, 429.9999999999999432, -244.9999999999999716 ) ) ;
#41293=EDGE_LOOP ( 'NONE', ( #42221, #13656, #14064, #16824 ) ) ;
#41510=LINE ( 'NONE', #23931, #3240 ) ;
#41669=CARTESIAN_POINT ( 'NONE',  ( 200.7583438952258916, 294.6698570112193920, -224.9999999999999716 ) ) ;
#42127=FACE_OUTER_BOUND ( 'NONE', #22217, .T. ) ;
#42212=VERTEX_POINT ( 'NONE', #2705 ) ;
#42221=ORIENTED_EDGE ( 'NONE', *, *, #34585, .T. ) ;
#42339=CARTESIAN_POINT ( 'NONE',  ( -180.7583438952261474, 1.505115564641941601E-13, -244.9999999999999716 ) ) ;
#42969=EDGE_CURVE ( 'NONE', #14164, #32232, #43992, .T. ) ;
#43050=CARTESIAN_POINT ( 'NONE',  ( -200.7583438952259485, 394.6698570112193920, -274.9999999999999432 ) ) ;
#43166=AXIS2_PLACEMENT_3D ( 'NONE', #20444, #38235, #20659 ) ;
#43387=ORIENTED_EDGE ( 'NONE', *, *, #12538, .F. ) ;
#43391=DIRECTION ( 'NONE',  ( 1.000000000000000000, 0.000000000000000000, 0.000000000000000000 ) ) ;
#43443=LINE ( 'NONE', #266, #10661 ) ;
#43514=ORIENTED_EDGE ( 'NONE', *, *, #30379, .T. ) ;
#43529=ORIENTED_EDGE ( 'NONE', *, *, #7822, .F. ) ;
#43534=DIRECTION ( 'NONE',  ( 8.326672684688676025E-16, -1.000000000000000000, 0.000000000000000000 ) ) ;
#43542=ADVANCED_FACE ( 'NONE', ( #42127 ), #17429, .F. ) ;
#43551=FACE_OUTER_BOUND ( 'NONE', #39970, .T. ) ;
#43622=CARTESIAN_POINT ( 'NONE',  ( 180.7583438952258916, 294.6698570112193920, -224.9999999999999716 ) ) ;
#43706=CARTESIAN_POINT ( 'NONE',  ( 180.7583438952259201, 294.6698570112193920, -244.9999999999999716 ) ) ;
#43738=ORIENTED_EDGE ( 'NONE', *, *, #5789, .F. ) ;
#43808=DIRECTION ( 'NONE',  ( 1.892425610156518354E-16, 1.000000000000000000, -0.000000000000000000 ) ) ;
#43867=VECTOR ( 'NONE', #2181, 1000.000000000000000 ) ;
#43935=FACE_BOUND ( 'NONE', #24529, .T. ) ;
#43972=ORIENTED_EDGE ( 'NONE', *, *, #44199, .T. ) ;
#43982=DIRECTION ( 'NONE',  ( 1.000000000000000000, 0.000000000000000000, 0.000000000000000000 ) ) ;
#43992=LINE ( 'NONE', #8685, #11296 ) ;
#44075=ORIENTED_EDGE ( 'NONE', *, *, #37114, .F. ) ;
#44199=EDGE_CURVE ( 'NONE', #4508, #42212, #17721, .T. ) ;
#44231=DIRECTION ( 'NONE',  ( -0.000000000000000000, -0.000000000000000000, 1.000000000000000000 ) ) ;
#44320=VERTEX_POINT ( 'NONE', #45673 ) ;
#44437=EDGE_LOOP ( 'NONE', ( #16538, #43529, #45333, #6063 ) ) ;
#44462=EDGE_CURVE ( 'NONE', #9555, #44320, #41510, .T. ) ;
#44518=PRODUCT_DEFINITION ( 'UNKNOWN', '', #12056, #20563 ) ;
#44536=ORIENTED_EDGE ( 'NONE', *, *, #21274, .T. ) ;
#44550=VECTOR ( 'NONE', #44231, 1000.000000000000000 ) ;
#44652=AXIS2_PLACEMENT_3D ( 'NONE', #39709, #35992, #32302 ) ;
#44679=EDGE_LOOP ( 'NONE', ( #39695, #29272, #3873, #11440 ) ) ;
#44817=CYLINDRICAL_SURFACE ( 'NONE', #40925, 10.00000000000000888 ) ;
#44906=ORIENTED_EDGE ( 'NONE', *, *, #6658, .F. ) ;
#45007=EDGE_CURVE ( 'NONE', #8754, #27855, #8451, .T. ) ;
#45008=ORIENTED_EDGE ( 'NONE', *, *, #4964, .T. ) ;
#45098=EDGE_CURVE ( 'NONE', #44320, #36156, #36632, .T. ) ;
#45108=( NAMED_UNIT ( * ) PLANE_ANGLE_UNIT ( ) SI_UNIT ( $, .RADIAN. ) );
#45277=EDGE_LOOP ( 'NONE', ( #16714, #38573, #27, #39055 ) ) ;
#45333=ORIENTED_EDGE ( 'NONE', *, *, #45098, .F. ) ;
#45366=VERTEX_POINT ( 'NONE', #38443 ) ;
#45401=VECTOR ( 'NONE', #21396, 1000.000000000000000 ) ;
#45518=VERTEX_POINT ( 'NONE', #20649 ) ;
#45626=LINE ( 'NONE', #20878, #5489 ) ;
#45673=CARTESIAN_POINT ( 'NONE',  ( -879.9999999999992042, 240.0000000000002274, -224.9999999999999716 ) ) ;
#45773=COLOUR_RGB('Off White',0.89,0.88,0.83);
#45774=FILL_AREA_STYLE_COLOUR('',#45773);
#45775=FILL_AREA_STYLE('',(#45774));
#45776=SURFACE_STYLE_FILL_AREA(#45775);
#45777=SURFACE_SIDE_STYLE('',(#45776));
#45778=SURFACE_STYLE_USAGE(.BOTH.,#45777);
#45779=PRESENTATION_STYLE_ASSIGNMENT((#45778));
ENDSEC;
END-ISO-10303-21;
